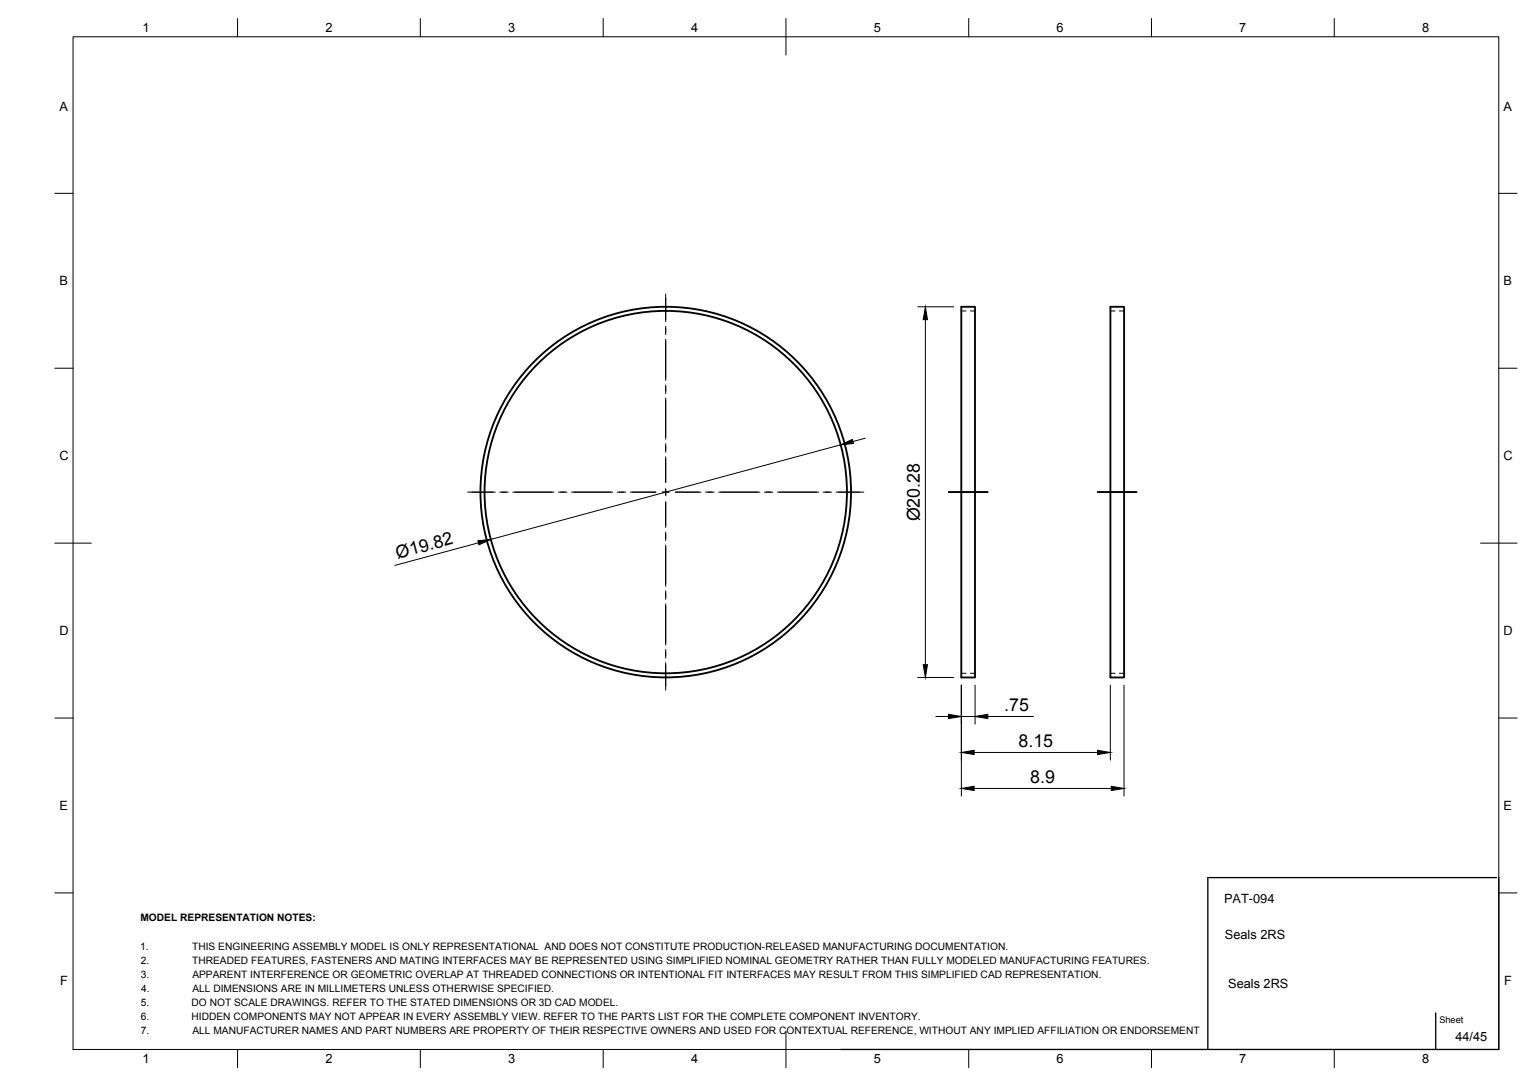
ISO-10303-21;
HEADER;
/* Generated by software containing ST-Developer
 * from STEP Tools, Inc. (www.steptools.com) 
 */

FILE_DESCRIPTION(
/* description */ ('Shaft runout checking stand'),
/* implementation_level */ '2;1');

FILE_NAME(
/* name */ 'Seals 2RS.step',
/* time_stamp */ '2026-11-02T21:12:33-08:00',
/* author */ (''),
/* organization */ (''),
/* preprocessor_version */ 'ST-DEVELOPER v20.2',
/* originating_system */ 'Autodesk Translation Framework v15.17.0.0',
/* authorisation */ '');

FILE_SCHEMA (('AUTOMOTIVE_DESIGN { 1 0 10303 214 3 1 1 }'));
ENDSEC;

DATA;
#10=MECHANICAL_DESIGN_GEOMETRIC_PRESENTATION_REPRESENTATION('',(#509,#510),#11748);
#416=SHAPE_REPRESENTATION_RELATIONSHIP('SRR','None',#11968,#459);
#459=ADVANCED_BREP_SHAPE_REPRESENTATION('',(#557,#558),#11744);
#509=STYLED_ITEM('',(#12169),#557);
#510=STYLED_ITEM('',(#12169),#558);
#557=MANIFOLD_SOLID_BREP('Body1',#6255);
#558=MANIFOLD_SOLID_BREP('Body2',#6256);
#663=FACE_BOUND('',#1856,.T.);
#664=FACE_BOUND('',#1859,.T.);
#665=FACE_BOUND('',#1862,.T.);
#666=FACE_BOUND('',#1865,.T.);
#918=CIRCLE('',#7435,1.013815);
#919=CIRCLE('',#7436,0.991185);
#920=CIRCLE('',#7438,1.013815);
#921=CIRCLE('',#7440,0.991185);
#922=CIRCLE('',#7443,1.013815);
#923=CIRCLE('',#7444,0.991185);
#924=CIRCLE('',#7446,1.013815);
#925=CIRCLE('',#7448,0.991185);
#1028=CYLINDRICAL_SURFACE('',#7437,1.013815);
#1029=CYLINDRICAL_SURFACE('',#7441,0.991185);
#1030=CYLINDRICAL_SURFACE('',#7445,1.013815);
#1031=CYLINDRICAL_SURFACE('',#7449,0.991185);
#1386=FACE_OUTER_BOUND('',#1855,.T.);
#1387=FACE_OUTER_BOUND('',#1857,.T.);
#1388=FACE_OUTER_BOUND('',#1858,.T.);
#1389=FACE_OUTER_BOUND('',#1860,.T.);
#1390=FACE_OUTER_BOUND('',#1861,.T.);
#1391=FACE_OUTER_BOUND('',#1863,.T.);
#1392=FACE_OUTER_BOUND('',#1864,.T.);
#1393=FACE_OUTER_BOUND('',#1866,.T.);
#1855=EDGE_LOOP('',(#5544));
#1856=EDGE_LOOP('',(#5545));
#1857=EDGE_LOOP('',(#5546,#5547,#5548,#5549));
#1858=EDGE_LOOP('',(#5550));
#1859=EDGE_LOOP('',(#5551));
#1860=EDGE_LOOP('',(#5552,#5553,#5554,#5555));
#1861=EDGE_LOOP('',(#5556));
#1862=EDGE_LOOP('',(#5557));
#1863=EDGE_LOOP('',(#5558,#5559,#5560,#5561));
#1864=EDGE_LOOP('',(#5562));
#1865=EDGE_LOOP('',(#5563));
#1866=EDGE_LOOP('',(#5564,#5565,#5566,#5567));
#2342=LINE('',#11571,#2809);
#2343=LINE('',#11576,#2810);
#2344=LINE('',#11585,#2811);
#2345=LINE('',#11590,#2812);
#2809=VECTOR('',#9359,1.013815);
#2810=VECTOR('',#9366,0.991185);
#2811=VECTOR('',#9377,1.013815);
#2812=VECTOR('',#9384,0.991185);
#3310=VERTEX_POINT('',#11564);
#3311=VERTEX_POINT('',#11566);
#3312=VERTEX_POINT('',#11569);
#3313=VERTEX_POINT('',#11573);
#3314=VERTEX_POINT('',#11578);
#3315=VERTEX_POINT('',#11580);
#3316=VERTEX_POINT('',#11583);
#3317=VERTEX_POINT('',#11587);
#4058=EDGE_CURVE('',#3310,#3310,#918,.T.);
#4059=EDGE_CURVE('',#3311,#3311,#919,.T.);
#4060=EDGE_CURVE('',#3312,#3312,#920,.T.);
#4061=EDGE_CURVE('',#3312,#3310,#2342,.T.);
#4062=EDGE_CURVE('',#3313,#3313,#921,.T.);
#4063=EDGE_CURVE('',#3313,#3311,#2343,.T.);
#4064=EDGE_CURVE('',#3314,#3314,#922,.T.);
#4065=EDGE_CURVE('',#3315,#3315,#923,.T.);
#4066=EDGE_CURVE('',#3316,#3316,#924,.T.);
#4067=EDGE_CURVE('',#3316,#3314,#2344,.T.);
#4068=EDGE_CURVE('',#3317,#3317,#925,.T.);
#4069=EDGE_CURVE('',#3317,#3315,#2345,.T.);
#5544=ORIENTED_EDGE('',*,*,#4058,.F.);
#5545=ORIENTED_EDGE('',*,*,#4059,.T.);
#5546=ORIENTED_EDGE('',*,*,#4060,.F.);
#5547=ORIENTED_EDGE('',*,*,#4061,.T.);
#5548=ORIENTED_EDGE('',*,*,#4058,.T.);
#5549=ORIENTED_EDGE('',*,*,#4061,.F.);
#5550=ORIENTED_EDGE('',*,*,#4060,.T.);
#5551=ORIENTED_EDGE('',*,*,#4062,.F.);
#5552=ORIENTED_EDGE('',*,*,#4062,.T.);
#5553=ORIENTED_EDGE('',*,*,#4063,.T.);
#5554=ORIENTED_EDGE('',*,*,#4059,.F.);
#5555=ORIENTED_EDGE('',*,*,#4063,.F.);
#5556=ORIENTED_EDGE('',*,*,#4064,.F.);
#5557=ORIENTED_EDGE('',*,*,#4065,.T.);
#5558=ORIENTED_EDGE('',*,*,#4066,.F.);
#5559=ORIENTED_EDGE('',*,*,#4067,.T.);
#5560=ORIENTED_EDGE('',*,*,#4064,.T.);
#5561=ORIENTED_EDGE('',*,*,#4067,.F.);
#5562=ORIENTED_EDGE('',*,*,#4066,.T.);
#5563=ORIENTED_EDGE('',*,*,#4068,.F.);
#5564=ORIENTED_EDGE('',*,*,#4068,.T.);
#5565=ORIENTED_EDGE('',*,*,#4069,.T.);
#5566=ORIENTED_EDGE('',*,*,#4065,.F.);
#5567=ORIENTED_EDGE('',*,*,#4069,.F.);
#5828=PLANE('',#7434);
#5829=PLANE('',#7439);
#5830=PLANE('',#7442);
#5831=PLANE('',#7447);
#6186=ADVANCED_FACE('',(#1386,#663),#5828,.T.);
#6187=ADVANCED_FACE('',(#1387),#1028,.T.);
#6188=ADVANCED_FACE('',(#1388,#664),#5829,.T.);
#6189=ADVANCED_FACE('',(#1389),#1029,.F.);
#6190=ADVANCED_FACE('',(#1390,#665),#5830,.T.);
#6191=ADVANCED_FACE('',(#1391),#1030,.T.);
#6192=ADVANCED_FACE('',(#1392,#666),#5831,.T.);
#6193=ADVANCED_FACE('',(#1393),#1031,.F.);
#6255=CLOSED_SHELL('',(#6186,#6187,#6188,#6189));
#6256=CLOSED_SHELL('',(#6190,#6191,#6192,#6193));
#7433=AXIS2_PLACEMENT_3D('',#11562,#9347,#9348);
#7434=AXIS2_PLACEMENT_3D('',#11563,#9349,#9350);
#7435=AXIS2_PLACEMENT_3D('',#11565,#9351,#9352);
#7436=AXIS2_PLACEMENT_3D('',#11567,#9353,#9354);
#7437=AXIS2_PLACEMENT_3D('',#11568,#9355,#9356);
#7438=AXIS2_PLACEMENT_3D('',#11570,#9357,#9358);
#7439=AXIS2_PLACEMENT_3D('',#11572,#9360,#9361);
#7440=AXIS2_PLACEMENT_3D('',#11574,#9362,#9363);
#7441=AXIS2_PLACEMENT_3D('',#11575,#9364,#9365);
#7442=AXIS2_PLACEMENT_3D('',#11577,#9367,#9368);
#7443=AXIS2_PLACEMENT_3D('',#11579,#9369,#9370);
#7444=AXIS2_PLACEMENT_3D('',#11581,#9371,#9372);
#7445=AXIS2_PLACEMENT_3D('',#11582,#9373,#9374);
#7446=AXIS2_PLACEMENT_3D('',#11584,#9375,#9376);
#7447=AXIS2_PLACEMENT_3D('',#11586,#9378,#9379);
#7448=AXIS2_PLACEMENT_3D('',#11588,#9380,#9381);
#7449=AXIS2_PLACEMENT_3D('',#11589,#9382,#9383);
#9347=DIRECTION('axis',(0.,0.,1.));
#9348=DIRECTION('refdir',(1.,0.,0.));
#9349=DIRECTION('center_axis',(0.,1.,0.));
#9350=DIRECTION('ref_axis',(0.,0.,1.));
#9351=DIRECTION('center_axis',(0.,-1.,0.));
#9352=DIRECTION('ref_axis',(1.,0.,0.));
#9353=DIRECTION('center_axis',(0.,-1.,0.));
#9354=DIRECTION('ref_axis',(1.,0.,0.));
#9355=DIRECTION('center_axis',(0.,-1.,0.));
#9356=DIRECTION('ref_axis',(1.,0.,0.));
#9357=DIRECTION('center_axis',(0.,-1.,0.));
#9358=DIRECTION('ref_axis',(1.,0.,0.));
#9359=DIRECTION('',(0.,1.,0.));
#9360=DIRECTION('center_axis',(0.,-1.,0.));
#9361=DIRECTION('ref_axis',(0.,0.,-1.));
#9362=DIRECTION('center_axis',(0.,-1.,0.));
#9363=DIRECTION('ref_axis',(1.,0.,0.));
#9364=DIRECTION('center_axis',(0.,-1.,0.));
#9365=DIRECTION('ref_axis',(1.,0.,0.));
#9366=DIRECTION('',(0.,1.,0.));
#9367=DIRECTION('center_axis',(0.,1.,0.));
#9368=DIRECTION('ref_axis',(0.,0.,1.));
#9369=DIRECTION('center_axis',(0.,-1.,0.));
#9370=DIRECTION('ref_axis',(1.,0.,0.));
#9371=DIRECTION('center_axis',(0.,-1.,0.));
#9372=DIRECTION('ref_axis',(1.,0.,0.));
#9373=DIRECTION('center_axis',(0.,-1.,0.));
#9374=DIRECTION('ref_axis',(1.,0.,0.));
#9375=DIRECTION('center_axis',(0.,-1.,0.));
#9376=DIRECTION('ref_axis',(1.,0.,0.));
#9377=DIRECTION('',(0.,1.,0.));
#9378=DIRECTION('center_axis',(0.,-1.,0.));
#9379=DIRECTION('ref_axis',(0.,0.,-1.));
#9380=DIRECTION('center_axis',(0.,-1.,0.));
#9381=DIRECTION('ref_axis',(1.,0.,0.));
#9382=DIRECTION('center_axis',(0.,-1.,0.));
#9383=DIRECTION('ref_axis',(1.,0.,0.));
#9384=DIRECTION('',(0.,1.,0.));
#11562=CARTESIAN_POINT('',(0.,0.,0.));
#11563=CARTESIAN_POINT('Origin',(1.013815,0.445,0.));
#11564=CARTESIAN_POINT('',(-1.013815,0.445,-1.24156529467757E-16));
#11565=CARTESIAN_POINT('Origin',(0.,0.445,0.));
#11566=CARTESIAN_POINT('',(-0.991185,0.445,-1.21385153761287E-16));
#11567=CARTESIAN_POINT('Origin',(0.,0.445,0.));
#11568=CARTESIAN_POINT('Origin',(0.,0.4075,0.));
#11569=CARTESIAN_POINT('',(-1.013815,0.37,-1.24156529467757E-16));
#11570=CARTESIAN_POINT('Origin',(0.,0.37,0.));
#11571=CARTESIAN_POINT('',(-1.013815,0.4075,-1.24156529467757E-16));
#11572=CARTESIAN_POINT('Origin',(0.991185,0.37,0.));
#11573=CARTESIAN_POINT('',(-0.991185,0.37,-1.21385153761287E-16));
#11574=CARTESIAN_POINT('Origin',(0.,0.37,0.));
#11575=CARTESIAN_POINT('Origin',(0.,0.4075,0.));
#11576=CARTESIAN_POINT('',(-0.991185,0.4075,-1.21385153761287E-16));
#11577=CARTESIAN_POINT('Origin',(1.013815,-0.37,0.));
#11578=CARTESIAN_POINT('',(-1.013815,-0.37,-1.24156529467757E-16));
#11579=CARTESIAN_POINT('Origin',(0.,-0.37,0.));
#11580=CARTESIAN_POINT('',(-0.991185,-0.37,-1.21385153761287E-16));
#11581=CARTESIAN_POINT('Origin',(0.,-0.37,0.));
#11582=CARTESIAN_POINT('Origin',(0.,-0.4075,0.));
#11583=CARTESIAN_POINT('',(-1.013815,-0.445,-1.24156529467757E-16));
#11584=CARTESIAN_POINT('Origin',(0.,-0.445,0.));
#11585=CARTESIAN_POINT('',(-1.013815,-0.4075,-1.24156529467757E-16));
#11586=CARTESIAN_POINT('Origin',(0.991185,-0.445,0.));
#11587=CARTESIAN_POINT('',(-0.991185,-0.445,-1.21385153761287E-16));
#11588=CARTESIAN_POINT('Origin',(0.,-0.445,0.));
#11589=CARTESIAN_POINT('Origin',(0.,-0.4075,0.));
#11590=CARTESIAN_POINT('',(-0.991185,-0.4075,-1.21385153761287E-16));
#11695=UNCERTAINTY_MEASURE_WITH_UNIT(LENGTH_MEASURE(0.001),#11749,
'DISTANCE_ACCURACY_VALUE',
'Maximum model space distance between geometric entities at asserted c
onnectivities');
#11699=UNCERTAINTY_MEASURE_WITH_UNIT(LENGTH_MEASURE(0.001),#11749,
'DISTANCE_ACCURACY_VALUE',
'Maximum model space distance between geometric entities at asserted c
onnectivities');
#11744=(
GEOMETRIC_REPRESENTATION_CONTEXT(3)
GLOBAL_UNCERTAINTY_ASSIGNED_CONTEXT((#11695))
GLOBAL_UNIT_ASSIGNED_CONTEXT((#11749,#11751,#11752))
REPRESENTATION_CONTEXT('','3D')
);
#11748=(
GEOMETRIC_REPRESENTATION_CONTEXT(3)
GLOBAL_UNCERTAINTY_ASSIGNED_CONTEXT((#11699))
GLOBAL_UNIT_ASSIGNED_CONTEXT((#11749,#11751,#11752))
REPRESENTATION_CONTEXT('','3D')
);
#11749=(
LENGTH_UNIT()
NAMED_UNIT(*)
SI_UNIT(.CENTI.,.METRE.)
);
#11751=(
NAMED_UNIT(*)
PLANE_ANGLE_UNIT()
SI_UNIT($,.RADIAN.)
);
#11752=(
NAMED_UNIT(*)
SI_UNIT($,.STERADIAN.)
SOLID_ANGLE_UNIT()
);
#11797=SHAPE_DEFINITION_REPRESENTATION(#11905,#11968);
#11905=PRODUCT_DEFINITION_SHAPE('',$,#12017);
#11968=SHAPE_REPRESENTATION('',(#7433),#11744);
#11972=PRODUCT_DEFINITION_CONTEXT('part definition',#12118,'design');
#12017=PRODUCT_DEFINITION('Seals 2RS','Seals 2RS',#12065,#11972);
#12065=PRODUCT_DEFINITION_FORMATION('',$,#12164);
#12118=APPLICATION_CONTEXT(
'Core Data for Automotive Mechanical Design Process');
#12119=PRODUCT_CONTEXT('part definition',#12118,'mechanical');
#12164=PRODUCT('Seals 2RS','Seals 2RS','Seals 2RS',(#12119));
#12169=PRESENTATION_STYLE_ASSIGNMENT((#12174));
#12174=SURFACE_STYLE_USAGE(.BOTH.,#12179);
#12179=SURFACE_SIDE_STYLE('',(#12184));
#12184=SURFACE_STYLE_FILL_AREA(#12189);
#12189=FILL_AREA_STYLE('CAD Library Painted - Engineering blue',(#12194));
#12194=FILL_AREA_STYLE_COLOUR('CAD Library Painted - Engineering blue',
#12199);
#12199=COLOUR_RGB('CAD Library Painted - Engineering blue',0.12156862745098,
0.356862745098039,0.6);
ENDSEC;
END-ISO-10303-21;
